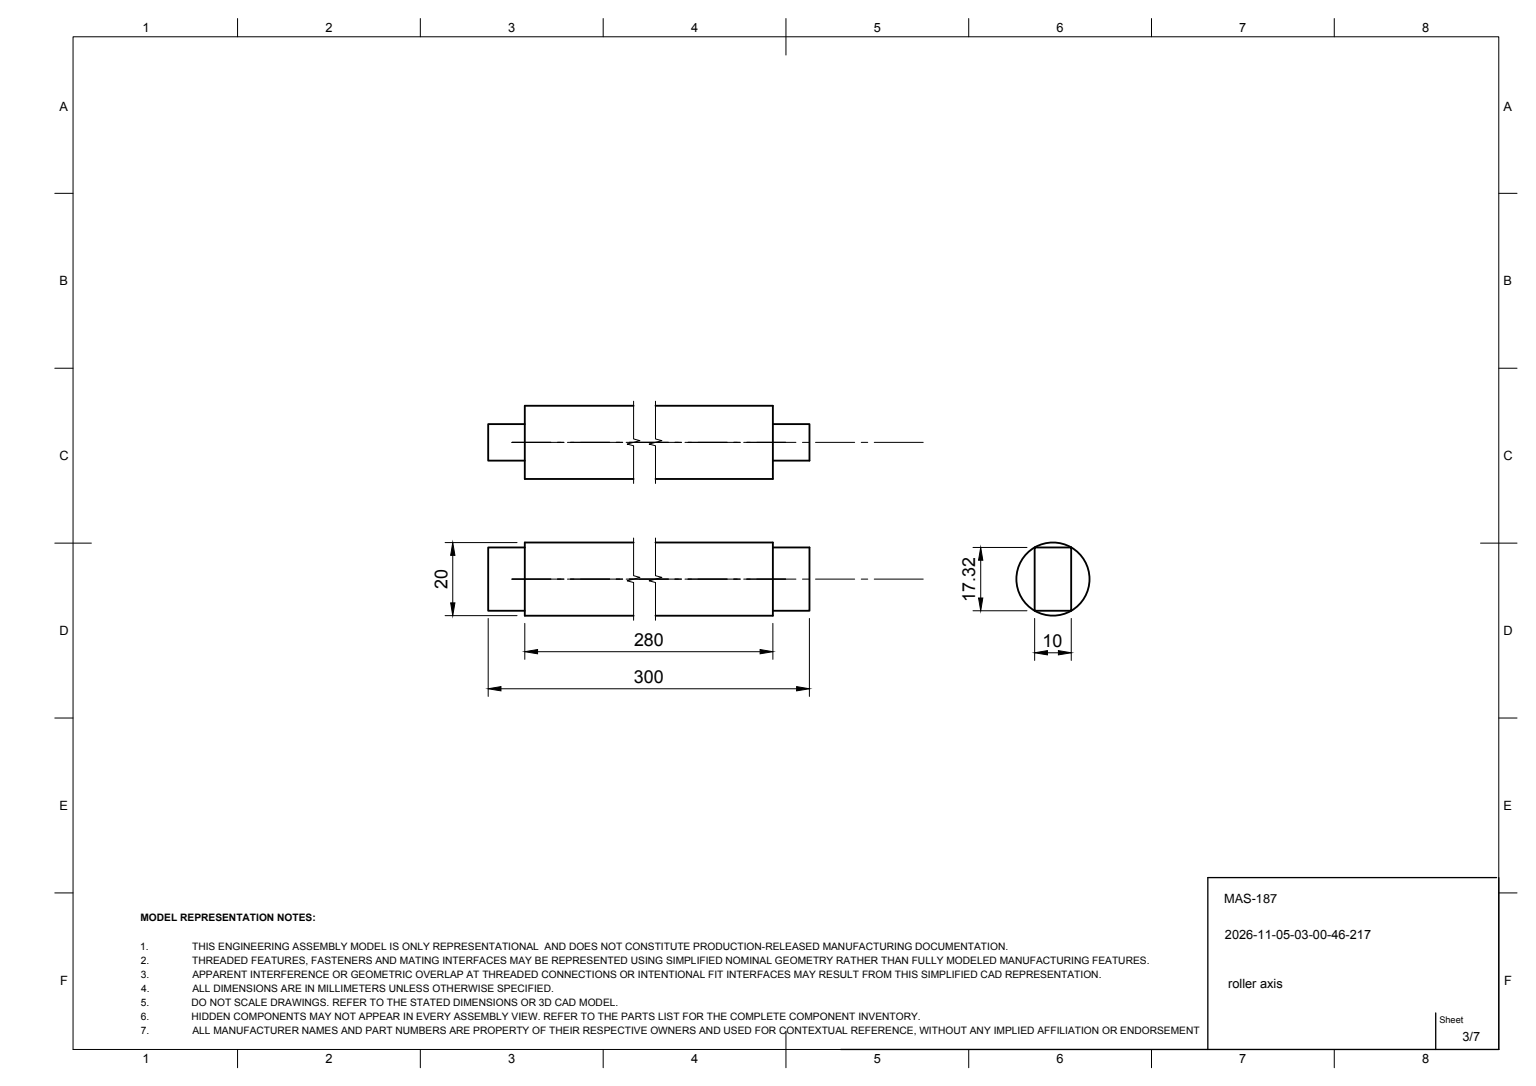
ISO-10303-21;
HEADER;
/* Generated by software containing ST-Developer
 * from STEP Tools, Inc. (www.steptools.com) 
 */

FILE_DESCRIPTION(
/* description */ ('STEP AP214'),
/* implementation_level */ '2;1');

FILE_NAME(
/* name */ 'roller axis.step',
/* time_stamp */ '2026-11-04T19:00:26-08:00',
/* author */ (''),
/* organization */ (''),
/* preprocessor_version */ 'ST-DEVELOPER v20.2',
/* originating_system */ 'Autodesk Translation Framework v15.17.0.0',
/* authorisation */ '');

FILE_SCHEMA (('AUTOMOTIVE_DESIGN { 1 0 10303 214 3 1 1 }'));
ENDSEC;

DATA;
#10=MECHANICAL_DESIGN_GEOMETRIC_PRESENTATION_REPRESENTATION('',(#273),#5689);
#259=SHAPE_REPRESENTATION_RELATIONSHIP('SRR','None',#5760,#266);
#266=ADVANCED_BREP_SHAPE_REPRESENTATION('',(#280),#5684);
#273=STYLED_ITEM('',(#5804),#280);
#280=MANIFOLD_SOLID_BREP('Body1',#2963);
#393=PLANE('',#3168);
#394=PLANE('',#3169);
#395=PLANE('',#3170);
#396=PLANE('',#3171);
#397=PLANE('',#3172);
#398=PLANE('',#3173);
#399=PLANE('',#3174);
#400=PLANE('',#3175);
#401=PLANE('',#3176);
#402=PLANE('',#3177);
#403=PLANE('',#3178);
#404=PLANE('',#3179);
#405=PLANE('',#3180);
#406=PLANE('',#3181);
#407=PLANE('',#3182);
#408=PLANE('',#3183);
#409=PLANE('',#3184);
#410=PLANE('',#3185);
#511=FACE_OUTER_BOUND('',#716,.T.);
#512=FACE_OUTER_BOUND('',#717,.T.);
#513=FACE_OUTER_BOUND('',#718,.T.);
#514=FACE_OUTER_BOUND('',#719,.T.);
#515=FACE_OUTER_BOUND('',#720,.T.);
#516=FACE_OUTER_BOUND('',#721,.T.);
#517=FACE_OUTER_BOUND('',#722,.T.);
#518=FACE_OUTER_BOUND('',#723,.T.);
#519=FACE_OUTER_BOUND('',#724,.T.);
#520=FACE_OUTER_BOUND('',#725,.T.);
#521=FACE_OUTER_BOUND('',#726,.T.);
#522=FACE_OUTER_BOUND('',#727,.T.);
#523=FACE_OUTER_BOUND('',#728,.T.);
#524=FACE_OUTER_BOUND('',#729,.T.);
#525=FACE_OUTER_BOUND('',#730,.T.);
#526=FACE_OUTER_BOUND('',#731,.T.);
#527=FACE_OUTER_BOUND('',#732,.T.);
#528=FACE_OUTER_BOUND('',#733,.T.);
#529=FACE_OUTER_BOUND('',#734,.T.);
#716=EDGE_LOOP('',(#2402,#2403,#2404,#2405,#2406,#2407,#2408,#2409,#2410,
#2411,#2412,#2413));
#717=EDGE_LOOP('',(#2414,#2415,#2416));
#718=EDGE_LOOP('',(#2417,#2418));
#719=EDGE_LOOP('',(#2419,#2420));
#720=EDGE_LOOP('',(#2421,#2422));
#721=EDGE_LOOP('',(#2423,#2424,#2425));
#722=EDGE_LOOP('',(#2426,#2427));
#723=EDGE_LOOP('',(#2428,#2429));
#724=EDGE_LOOP('',(#2430,#2431));
#725=EDGE_LOOP('',(#2432,#2433,#2434,#2435));
#726=EDGE_LOOP('',(#2436,#2437,#2438,#2439));
#727=EDGE_LOOP('',(#2440,#2441,#2442,#2443));
#728=EDGE_LOOP('',(#2444,#2445,#2446,#2447));
#729=EDGE_LOOP('',(#2448,#2449,#2450,#2451));
#730=EDGE_LOOP('',(#2452,#2453,#2454,#2455));
#731=EDGE_LOOP('',(#2456,#2457,#2458,#2459));
#732=EDGE_LOOP('',(#2460,#2461,#2462,#2463));
#733=EDGE_LOOP('',(#2464,#2465,#2466,#2467));
#734=EDGE_LOOP('',(#2468,#2469,#2470,#2471));
#975=LINE('',#4653,#1206);
#976=LINE('',#4667,#1207);
#977=LINE('',#4669,#1208);
#978=LINE('',#4671,#1209);
#979=LINE('',#4673,#1210);
#980=LINE('',#4675,#1211);
#981=LINE('',#4677,#1212);
#982=LINE('',#4679,#1213);
#983=LINE('',#4681,#1214);
#984=LINE('',#4685,#1215);
#985=LINE('',#4687,#1216);
#986=LINE('',#4689,#1217);
#987=LINE('',#4690,#1218);
#988=LINE('',#4692,#1219);
#989=LINE('',#4693,#1220);
#990=LINE('',#4695,#1221);
#991=LINE('',#4697,#1222);
#992=LINE('',#4701,#1223);
#993=LINE('',#4703,#1224);
#994=LINE('',#4704,#1225);
#995=LINE('',#4707,#1226);
#996=LINE('',#4708,#1227);
#997=LINE('',#4711,#1228);
#998=LINE('',#4712,#1229);
#999=LINE('',#4714,#1230);
#1206=VECTOR('',#3756,10.);
#1207=VECTOR('',#3773,1000.);
#1208=VECTOR('',#3776,1000.);
#1209=VECTOR('',#3779,1000.);
#1210=VECTOR('',#3782,1000.);
#1211=VECTOR('',#3785,1000.);
#1212=VECTOR('',#3788,1000.);
#1213=VECTOR('',#3791,1000.);
#1214=VECTOR('',#3794,1000.);
#1215=VECTOR('',#3797,1000.);
#1216=VECTOR('',#3798,1000.);
#1217=VECTOR('',#3799,1000.);
#1218=VECTOR('',#3800,1000.);
#1219=VECTOR('',#3803,1000.);
#1220=VECTOR('',#3804,1000.);
#1221=VECTOR('',#3807,1000.);
#1222=VECTOR('',#3810,1000.);
#1223=VECTOR('',#3815,1000.);
#1224=VECTOR('',#3816,1000.);
#1225=VECTOR('',#3817,1000.);
#1226=VECTOR('',#3820,1000.);
#1227=VECTOR('',#3821,1000.);
#1228=VECTOR('',#3824,1000.);
#1229=VECTOR('',#3825,1000.);
#1230=VECTOR('',#3828,1000.);
#1318=CIRCLE('',#3158,10.);
#1319=CIRCLE('',#3159,10.);
#1320=CIRCLE('',#3160,10.);
#1321=CIRCLE('',#3161,10.);
#1322=CIRCLE('',#3162,10.);
#1323=CIRCLE('',#3163,10.);
#1324=CIRCLE('',#3164,10.);
#1325=CIRCLE('',#3165,10.);
#1326=CIRCLE('',#3166,10.);
#1327=CIRCLE('',#3167,10.);
#1525=VERTEX_POINT('',#4645);
#1526=VERTEX_POINT('',#4646);
#1527=VERTEX_POINT('',#4648);
#1528=VERTEX_POINT('',#4650);
#1529=VERTEX_POINT('',#4652);
#1530=VERTEX_POINT('',#4654);
#1531=VERTEX_POINT('',#4656);
#1532=VERTEX_POINT('',#4658);
#1533=VERTEX_POINT('',#4660);
#1534=VERTEX_POINT('',#4663);
#1535=VERTEX_POINT('',#4683);
#1536=VERTEX_POINT('',#4684);
#1537=VERTEX_POINT('',#4686);
#1538=VERTEX_POINT('',#4688);
#1539=VERTEX_POINT('',#4700);
#1540=VERTEX_POINT('',#4702);
#1541=VERTEX_POINT('',#4706);
#1542=VERTEX_POINT('',#4710);
#1829=EDGE_CURVE('',#1525,#1526,#1318,.T.);
#1830=EDGE_CURVE('',#1526,#1527,#1319,.T.);
#1831=EDGE_CURVE('',#1527,#1528,#1320,.T.);
#1832=EDGE_CURVE('',#1528,#1529,#975,.T.);
#1833=EDGE_CURVE('',#1530,#1529,#1321,.T.);
#1834=EDGE_CURVE('',#1531,#1530,#1322,.T.);
#1835=EDGE_CURVE('',#1532,#1531,#1323,.T.);
#1836=EDGE_CURVE('',#1533,#1532,#1324,.T.);
#1837=EDGE_CURVE('',#1529,#1533,#1325,.T.);
#1838=EDGE_CURVE('',#1528,#1534,#1326,.T.);
#1839=EDGE_CURVE('',#1534,#1525,#1327,.T.);
#1840=EDGE_CURVE('',#1533,#1530,#976,.T.);
#1841=EDGE_CURVE('',#1532,#1533,#977,.T.);
#1842=EDGE_CURVE('',#1531,#1532,#978,.T.);
#1843=EDGE_CURVE('',#1530,#1531,#979,.T.);
#1844=EDGE_CURVE('',#1534,#1527,#980,.T.);
#1845=EDGE_CURVE('',#1525,#1534,#981,.T.);
#1846=EDGE_CURVE('',#1526,#1525,#982,.T.);
#1847=EDGE_CURVE('',#1527,#1526,#983,.T.);
#1848=EDGE_CURVE('',#1535,#1536,#984,.T.);
#1849=EDGE_CURVE('',#1537,#1535,#985,.T.);
#1850=EDGE_CURVE('',#1538,#1537,#986,.T.);
#1851=EDGE_CURVE('',#1536,#1538,#987,.T.);
#1852=EDGE_CURVE('',#1527,#1535,#988,.T.);
#1853=EDGE_CURVE('',#1526,#1537,#989,.T.);
#1854=EDGE_CURVE('',#1525,#1538,#990,.T.);
#1855=EDGE_CURVE('',#1534,#1536,#991,.T.);
#1856=EDGE_CURVE('',#1539,#1533,#992,.T.);
#1857=EDGE_CURVE('',#1540,#1539,#993,.T.);
#1858=EDGE_CURVE('',#1540,#1530,#994,.T.);
#1859=EDGE_CURVE('',#1541,#1532,#995,.T.);
#1860=EDGE_CURVE('',#1539,#1541,#996,.T.);
#1861=EDGE_CURVE('',#1542,#1531,#997,.T.);
#1862=EDGE_CURVE('',#1541,#1542,#998,.T.);
#1863=EDGE_CURVE('',#1542,#1540,#999,.T.);
#2402=ORIENTED_EDGE('',*,*,#1829,.T.);
#2403=ORIENTED_EDGE('',*,*,#1830,.T.);
#2404=ORIENTED_EDGE('',*,*,#1831,.T.);
#2405=ORIENTED_EDGE('',*,*,#1832,.T.);
#2406=ORIENTED_EDGE('',*,*,#1833,.F.);
#2407=ORIENTED_EDGE('',*,*,#1834,.F.);
#2408=ORIENTED_EDGE('',*,*,#1835,.F.);
#2409=ORIENTED_EDGE('',*,*,#1836,.F.);
#2410=ORIENTED_EDGE('',*,*,#1837,.F.);
#2411=ORIENTED_EDGE('',*,*,#1832,.F.);
#2412=ORIENTED_EDGE('',*,*,#1838,.T.);
#2413=ORIENTED_EDGE('',*,*,#1839,.T.);
#2414=ORIENTED_EDGE('',*,*,#1833,.T.);
#2415=ORIENTED_EDGE('',*,*,#1837,.T.);
#2416=ORIENTED_EDGE('',*,*,#1840,.T.);
#2417=ORIENTED_EDGE('',*,*,#1836,.T.);
#2418=ORIENTED_EDGE('',*,*,#1841,.T.);
#2419=ORIENTED_EDGE('',*,*,#1835,.T.);
#2420=ORIENTED_EDGE('',*,*,#1842,.T.);
#2421=ORIENTED_EDGE('',*,*,#1834,.T.);
#2422=ORIENTED_EDGE('',*,*,#1843,.T.);
#2423=ORIENTED_EDGE('',*,*,#1844,.F.);
#2424=ORIENTED_EDGE('',*,*,#1838,.F.);
#2425=ORIENTED_EDGE('',*,*,#1831,.F.);
#2426=ORIENTED_EDGE('',*,*,#1845,.F.);
#2427=ORIENTED_EDGE('',*,*,#1839,.F.);
#2428=ORIENTED_EDGE('',*,*,#1846,.F.);
#2429=ORIENTED_EDGE('',*,*,#1829,.F.);
#2430=ORIENTED_EDGE('',*,*,#1847,.F.);
#2431=ORIENTED_EDGE('',*,*,#1830,.F.);
#2432=ORIENTED_EDGE('',*,*,#1848,.F.);
#2433=ORIENTED_EDGE('',*,*,#1849,.F.);
#2434=ORIENTED_EDGE('',*,*,#1850,.F.);
#2435=ORIENTED_EDGE('',*,*,#1851,.F.);
#2436=ORIENTED_EDGE('',*,*,#1852,.F.);
#2437=ORIENTED_EDGE('',*,*,#1847,.T.);
#2438=ORIENTED_EDGE('',*,*,#1853,.T.);
#2439=ORIENTED_EDGE('',*,*,#1849,.T.);
#2440=ORIENTED_EDGE('',*,*,#1853,.F.);
#2441=ORIENTED_EDGE('',*,*,#1846,.T.);
#2442=ORIENTED_EDGE('',*,*,#1854,.T.);
#2443=ORIENTED_EDGE('',*,*,#1850,.T.);
#2444=ORIENTED_EDGE('',*,*,#1854,.F.);
#2445=ORIENTED_EDGE('',*,*,#1845,.T.);
#2446=ORIENTED_EDGE('',*,*,#1855,.T.);
#2447=ORIENTED_EDGE('',*,*,#1851,.T.);
#2448=ORIENTED_EDGE('',*,*,#1855,.F.);
#2449=ORIENTED_EDGE('',*,*,#1844,.T.);
#2450=ORIENTED_EDGE('',*,*,#1852,.T.);
#2451=ORIENTED_EDGE('',*,*,#1848,.T.);
#2452=ORIENTED_EDGE('',*,*,#1840,.F.);
#2453=ORIENTED_EDGE('',*,*,#1856,.F.);
#2454=ORIENTED_EDGE('',*,*,#1857,.F.);
#2455=ORIENTED_EDGE('',*,*,#1858,.T.);
#2456=ORIENTED_EDGE('',*,*,#1841,.F.);
#2457=ORIENTED_EDGE('',*,*,#1859,.F.);
#2458=ORIENTED_EDGE('',*,*,#1860,.F.);
#2459=ORIENTED_EDGE('',*,*,#1856,.T.);
#2460=ORIENTED_EDGE('',*,*,#1842,.F.);
#2461=ORIENTED_EDGE('',*,*,#1861,.F.);
#2462=ORIENTED_EDGE('',*,*,#1862,.F.);
#2463=ORIENTED_EDGE('',*,*,#1859,.T.);
#2464=ORIENTED_EDGE('',*,*,#1843,.F.);
#2465=ORIENTED_EDGE('',*,*,#1858,.F.);
#2466=ORIENTED_EDGE('',*,*,#1863,.F.);
#2467=ORIENTED_EDGE('',*,*,#1861,.T.);
#2468=ORIENTED_EDGE('',*,*,#1857,.T.);
#2469=ORIENTED_EDGE('',*,*,#1860,.T.);
#2470=ORIENTED_EDGE('',*,*,#1862,.T.);
#2471=ORIENTED_EDGE('',*,*,#1863,.T.);
#2787=CYLINDRICAL_SURFACE('',#3157,10.);
#2871=ADVANCED_FACE('',(#511),#2787,.T.);
#2872=ADVANCED_FACE('',(#512),#393,.T.);
#2873=ADVANCED_FACE('',(#513),#394,.T.);
#2874=ADVANCED_FACE('',(#514),#395,.T.);
#2875=ADVANCED_FACE('',(#515),#396,.T.);
#2876=ADVANCED_FACE('',(#516),#397,.F.);
#2877=ADVANCED_FACE('',(#517),#398,.F.);
#2878=ADVANCED_FACE('',(#518),#399,.F.);
#2879=ADVANCED_FACE('',(#519),#400,.F.);
#2880=ADVANCED_FACE('',(#520),#401,.F.);
#2881=ADVANCED_FACE('',(#521),#402,.F.);
#2882=ADVANCED_FACE('',(#522),#403,.F.);
#2883=ADVANCED_FACE('',(#523),#404,.F.);
#2884=ADVANCED_FACE('',(#524),#405,.F.);
#2885=ADVANCED_FACE('',(#525),#406,.F.);
#2886=ADVANCED_FACE('',(#526),#407,.F.);
#2887=ADVANCED_FACE('',(#527),#408,.F.);
#2888=ADVANCED_FACE('',(#528),#409,.F.);
#2889=ADVANCED_FACE('',(#529),#410,.T.);
#2963=CLOSED_SHELL('',(#2871,#2872,#2873,#2874,#2875,#2876,#2877,#2878,
#2879,#2880,#2881,#2882,#2883,#2884,#2885,#2886,#2887,#2888,#2889));
#3156=AXIS2_PLACEMENT_3D('',#4643,#3746,#3747);
#3157=AXIS2_PLACEMENT_3D('',#4644,#3748,#3749);
#3158=AXIS2_PLACEMENT_3D('',#4647,#3750,#3751);
#3159=AXIS2_PLACEMENT_3D('',#4649,#3752,#3753);
#3160=AXIS2_PLACEMENT_3D('',#4651,#3754,#3755);
#3161=AXIS2_PLACEMENT_3D('',#4655,#3757,#3758);
#3162=AXIS2_PLACEMENT_3D('',#4657,#3759,#3760);
#3163=AXIS2_PLACEMENT_3D('',#4659,#3761,#3762);
#3164=AXIS2_PLACEMENT_3D('',#4661,#3763,#3764);
#3165=AXIS2_PLACEMENT_3D('',#4662,#3765,#3766);
#3166=AXIS2_PLACEMENT_3D('',#4664,#3767,#3768);
#3167=AXIS2_PLACEMENT_3D('',#4665,#3769,#3770);
#3168=AXIS2_PLACEMENT_3D('',#4666,#3771,#3772);
#3169=AXIS2_PLACEMENT_3D('',#4668,#3774,#3775);
#3170=AXIS2_PLACEMENT_3D('',#4670,#3777,#3778);
#3171=AXIS2_PLACEMENT_3D('',#4672,#3780,#3781);
#3172=AXIS2_PLACEMENT_3D('',#4674,#3783,#3784);
#3173=AXIS2_PLACEMENT_3D('',#4676,#3786,#3787);
#3174=AXIS2_PLACEMENT_3D('',#4678,#3789,#3790);
#3175=AXIS2_PLACEMENT_3D('',#4680,#3792,#3793);
#3176=AXIS2_PLACEMENT_3D('',#4682,#3795,#3796);
#3177=AXIS2_PLACEMENT_3D('',#4691,#3801,#3802);
#3178=AXIS2_PLACEMENT_3D('',#4694,#3805,#3806);
#3179=AXIS2_PLACEMENT_3D('',#4696,#3808,#3809);
#3180=AXIS2_PLACEMENT_3D('',#4698,#3811,#3812);
#3181=AXIS2_PLACEMENT_3D('',#4699,#3813,#3814);
#3182=AXIS2_PLACEMENT_3D('',#4705,#3818,#3819);
#3183=AXIS2_PLACEMENT_3D('',#4709,#3822,#3823);
#3184=AXIS2_PLACEMENT_3D('',#4713,#3826,#3827);
#3185=AXIS2_PLACEMENT_3D('',#4715,#3829,#3830);
#3746=DIRECTION('axis',(0.,0.,1.));
#3747=DIRECTION('refdir',(1.,0.,0.));
#3748=DIRECTION('center_axis',(0.,0.,-1.));
#3749=DIRECTION('ref_axis',(-1.,0.,0.));
#3750=DIRECTION('center_axis',(0.,0.,1.));
#3751=DIRECTION('ref_axis',(1.,0.,0.));
#3752=DIRECTION('center_axis',(0.,0.,1.));
#3753=DIRECTION('ref_axis',(1.,0.,0.));
#3754=DIRECTION('center_axis',(0.,0.,1.));
#3755=DIRECTION('ref_axis',(1.,0.,0.));
#3756=DIRECTION('',(0.,0.,1.));
#3757=DIRECTION('center_axis',(0.,0.,1.));
#3758=DIRECTION('ref_axis',(1.,0.,0.));
#3759=DIRECTION('center_axis',(0.,0.,1.));
#3760=DIRECTION('ref_axis',(1.,0.,0.));
#3761=DIRECTION('center_axis',(0.,0.,1.));
#3762=DIRECTION('ref_axis',(1.,0.,0.));
#3763=DIRECTION('center_axis',(0.,0.,1.));
#3764=DIRECTION('ref_axis',(1.,0.,0.));
#3765=DIRECTION('center_axis',(0.,0.,1.));
#3766=DIRECTION('ref_axis',(1.,0.,0.));
#3767=DIRECTION('center_axis',(0.,0.,1.));
#3768=DIRECTION('ref_axis',(1.,0.,0.));
#3769=DIRECTION('center_axis',(0.,0.,1.));
#3770=DIRECTION('ref_axis',(1.,0.,0.));
#3771=DIRECTION('center_axis',(0.,0.,1.));
#3772=DIRECTION('ref_axis',(1.,0.,0.));
#3773=DIRECTION('',(0.,-1.,0.));
#3774=DIRECTION('center_axis',(0.,0.,1.));
#3775=DIRECTION('ref_axis',(1.,0.,0.));
#3776=DIRECTION('',(1.,0.,0.));
#3777=DIRECTION('center_axis',(0.,0.,1.));
#3778=DIRECTION('ref_axis',(1.,0.,0.));
#3779=DIRECTION('',(0.,1.,0.));
#3780=DIRECTION('center_axis',(0.,0.,1.));
#3781=DIRECTION('ref_axis',(1.,0.,0.));
#3782=DIRECTION('',(-1.,0.,0.));
#3783=DIRECTION('center_axis',(0.,0.,1.));
#3784=DIRECTION('ref_axis',(1.,0.,0.));
#3785=DIRECTION('',(0.,-1.,0.));
#3786=DIRECTION('center_axis',(0.,0.,1.));
#3787=DIRECTION('ref_axis',(1.,0.,0.));
#3788=DIRECTION('',(1.,0.,0.));
#3789=DIRECTION('center_axis',(0.,0.,1.));
#3790=DIRECTION('ref_axis',(1.,0.,0.));
#3791=DIRECTION('',(0.,1.,0.));
#3792=DIRECTION('center_axis',(0.,0.,1.));
#3793=DIRECTION('ref_axis',(1.,0.,0.));
#3794=DIRECTION('',(-1.,0.,0.));
#3795=DIRECTION('center_axis',(0.,0.,1.));
#3796=DIRECTION('ref_axis',(1.,0.,0.));
#3797=DIRECTION('',(0.,1.,0.));
#3798=DIRECTION('',(1.,0.,0.));
#3799=DIRECTION('',(0.,-1.,0.));
#3800=DIRECTION('',(-1.,0.,0.));
#3801=DIRECTION('center_axis',(0.,1.,0.));
#3802=DIRECTION('ref_axis',(0.,0.,1.));
#3803=DIRECTION('',(0.,0.,-1.));
#3804=DIRECTION('',(0.,0.,-1.));
#3805=DIRECTION('center_axis',(1.,0.,0.));
#3806=DIRECTION('ref_axis',(0.,0.,-1.));
#3807=DIRECTION('',(0.,0.,-1.));
#3808=DIRECTION('center_axis',(0.,-1.,0.));
#3809=DIRECTION('ref_axis',(0.,0.,-1.));
#3810=DIRECTION('',(0.,0.,-1.));
#3811=DIRECTION('center_axis',(-1.,0.,0.));
#3812=DIRECTION('ref_axis',(0.,0.,1.));
#3813=DIRECTION('center_axis',(-1.,0.,0.));
#3814=DIRECTION('ref_axis',(0.,0.,1.));
#3815=DIRECTION('',(0.,0.,-1.));
#3816=DIRECTION('',(0.,1.,0.));
#3817=DIRECTION('',(0.,0.,-1.));
#3818=DIRECTION('center_axis',(0.,-1.,0.));
#3819=DIRECTION('ref_axis',(0.,0.,-1.));
#3820=DIRECTION('',(0.,0.,-1.));
#3821=DIRECTION('',(-1.,0.,0.));
#3822=DIRECTION('center_axis',(1.,0.,0.));
#3823=DIRECTION('ref_axis',(0.,0.,-1.));
#3824=DIRECTION('',(0.,0.,-1.));
#3825=DIRECTION('',(0.,-1.,0.));
#3826=DIRECTION('center_axis',(0.,1.,0.));
#3827=DIRECTION('ref_axis',(0.,0.,1.));
#3828=DIRECTION('',(1.,0.,0.));
#3829=DIRECTION('center_axis',(0.,0.,1.));
#3830=DIRECTION('ref_axis',(1.,0.,0.));
#4643=CARTESIAN_POINT('',(0.,0.,0.));
#4644=CARTESIAN_POINT('Origin',(0.,0.,140.));
#4645=CARTESIAN_POINT('',(-5.,8.66025403784439,-140.));
#4646=CARTESIAN_POINT('',(-5.,-8.66025403784439,-140.));
#4647=CARTESIAN_POINT('Origin',(0.,0.,-140.));
#4648=CARTESIAN_POINT('',(5.,-8.66025403784439,-140.));
#4649=CARTESIAN_POINT('Origin',(0.,0.,-140.));
#4650=CARTESIAN_POINT('',(10.,-1.22464679914735E-15,-140.));
#4651=CARTESIAN_POINT('Origin',(0.,0.,-140.));
#4652=CARTESIAN_POINT('',(10.,-1.22464679914735E-15,140.));
#4653=CARTESIAN_POINT('',(10.,-1.22464679914735E-15,140.));
#4654=CARTESIAN_POINT('',(5.,-8.66025403784439,140.));
#4655=CARTESIAN_POINT('Origin',(0.,0.,140.));
#4656=CARTESIAN_POINT('',(-5.,-8.66025403784439,140.));
#4657=CARTESIAN_POINT('Origin',(0.,0.,140.));
#4658=CARTESIAN_POINT('',(-5.,8.66025403784439,140.));
#4659=CARTESIAN_POINT('Origin',(0.,0.,140.));
#4660=CARTESIAN_POINT('',(5.,8.66025403784439,140.));
#4661=CARTESIAN_POINT('Origin',(0.,0.,140.));
#4662=CARTESIAN_POINT('Origin',(0.,0.,140.));
#4663=CARTESIAN_POINT('',(4.99999999999999,8.66025403784439,-140.));
#4664=CARTESIAN_POINT('Origin',(0.,0.,-140.));
#4665=CARTESIAN_POINT('Origin',(0.,0.,-140.));
#4666=CARTESIAN_POINT('Origin',(0.,0.,140.));
#4667=CARTESIAN_POINT('',(5.,0.,140.));
#4668=CARTESIAN_POINT('Origin',(0.,0.,140.));
#4669=CARTESIAN_POINT('',(0.,8.66025403784439,140.));
#4670=CARTESIAN_POINT('Origin',(0.,0.,140.));
#4671=CARTESIAN_POINT('',(-5.,0.,140.));
#4672=CARTESIAN_POINT('Origin',(0.,0.,140.));
#4673=CARTESIAN_POINT('',(0.,-8.66025403784439,140.));
#4674=CARTESIAN_POINT('Origin',(0.,0.,-140.));
#4675=CARTESIAN_POINT('',(5.,0.,-140.));
#4676=CARTESIAN_POINT('Origin',(0.,0.,-140.));
#4677=CARTESIAN_POINT('',(0.,8.66025403784439,-140.));
#4678=CARTESIAN_POINT('Origin',(0.,0.,-140.));
#4679=CARTESIAN_POINT('',(-5.,0.,-140.));
#4680=CARTESIAN_POINT('Origin',(0.,0.,-140.));
#4681=CARTESIAN_POINT('',(0.,-8.66025403784439,-140.));
#4682=CARTESIAN_POINT('Origin',(0.,0.,-150.));
#4683=CARTESIAN_POINT('',(5.,-8.66025403784439,-150.));
#4684=CARTESIAN_POINT('',(5.,8.66025403784439,-150.));
#4685=CARTESIAN_POINT('',(5.,8.66025403784439,-150.));
#4686=CARTESIAN_POINT('',(-5.,-8.66025403784439,-150.));
#4687=CARTESIAN_POINT('',(-5.,-8.66025403784439,-150.));
#4688=CARTESIAN_POINT('',(-5.,8.66025403784439,-150.));
#4689=CARTESIAN_POINT('',(-5.,8.66025403784439,-150.));
#4690=CARTESIAN_POINT('',(-5.,8.66025403784439,-150.));
#4691=CARTESIAN_POINT('Origin',(-5.,-8.66025403784439,150.));
#4692=CARTESIAN_POINT('',(5.,-8.66025403784439,150.));
#4693=CARTESIAN_POINT('',(-5.,-8.66025403784439,150.));
#4694=CARTESIAN_POINT('Origin',(-5.,8.66025403784439,150.));
#4695=CARTESIAN_POINT('',(-5.,8.66025403784439,150.));
#4696=CARTESIAN_POINT('Origin',(-5.,8.66025403784439,150.));
#4697=CARTESIAN_POINT('',(5.,8.66025403784439,150.));
#4698=CARTESIAN_POINT('Origin',(5.,8.66025403784439,150.));
#4699=CARTESIAN_POINT('Origin',(5.,8.66025403784439,150.));
#4700=CARTESIAN_POINT('',(5.,8.66025403784439,150.));
#4701=CARTESIAN_POINT('',(5.,8.66025403784439,150.));
#4702=CARTESIAN_POINT('',(5.,-8.66025403784439,150.));
#4703=CARTESIAN_POINT('',(5.,8.66025403784439,150.));
#4704=CARTESIAN_POINT('',(5.,-8.66025403784439,150.));
#4705=CARTESIAN_POINT('Origin',(-5.,8.66025403784439,150.));
#4706=CARTESIAN_POINT('',(-5.,8.66025403784439,150.));
#4707=CARTESIAN_POINT('',(-5.,8.66025403784439,150.));
#4708=CARTESIAN_POINT('',(-5.,8.66025403784439,150.));
#4709=CARTESIAN_POINT('Origin',(-5.,8.66025403784439,150.));
#4710=CARTESIAN_POINT('',(-5.,-8.66025403784439,150.));
#4711=CARTESIAN_POINT('',(-5.,-8.66025403784439,150.));
#4712=CARTESIAN_POINT('',(-5.,8.66025403784439,150.));
#4713=CARTESIAN_POINT('Origin',(-5.,-8.66025403784439,150.));
#4714=CARTESIAN_POINT('',(-5.,-8.66025403784439,150.));
#4715=CARTESIAN_POINT('Origin',(0.,0.,150.));
#5675=UNCERTAINTY_MEASURE_WITH_UNIT(LENGTH_MEASURE(0.01),#5690,
'DISTANCE_ACCURACY_VALUE',
'Maximum model space distance between geometric entities at asserted c
onnectivities');
#5680=UNCERTAINTY_MEASURE_WITH_UNIT(LENGTH_MEASURE(0.01),#5690,
'DISTANCE_ACCURACY_VALUE',
'Maximum model space distance between geometric entities at asserted c
onnectivities');
#5684=(
GEOMETRIC_REPRESENTATION_CONTEXT(3)
GLOBAL_UNCERTAINTY_ASSIGNED_CONTEXT((#5675))
GLOBAL_UNIT_ASSIGNED_CONTEXT((#5690,#5692,#5693))
REPRESENTATION_CONTEXT('','3D')
);
#5689=(
GEOMETRIC_REPRESENTATION_CONTEXT(3)
GLOBAL_UNCERTAINTY_ASSIGNED_CONTEXT((#5680))
GLOBAL_UNIT_ASSIGNED_CONTEXT((#5690,#5692,#5693))
REPRESENTATION_CONTEXT('','3D')
);
#5690=(
LENGTH_UNIT()
NAMED_UNIT(*)
SI_UNIT(.MILLI.,.METRE.)
);
#5692=(
NAMED_UNIT(*)
PLANE_ANGLE_UNIT()
SI_UNIT($,.RADIAN.)
);
#5693=(
NAMED_UNIT(*)
SI_UNIT($,.STERADIAN.)
SOLID_ANGLE_UNIT()
);
#5697=SHAPE_DEFINITION_REPRESENTATION(#5705,#5760);
#5705=PRODUCT_DEFINITION_SHAPE('',$,#5769);
#5760=SHAPE_REPRESENTATION('',(#3156),#5684);
#5765=PRODUCT_DEFINITION_CONTEXT('part definition',#5791,'design');
#5769=PRODUCT_DEFINITION('roller axis','roller axis',#5777,#5765);
#5777=PRODUCT_DEFINITION_FORMATION('',$,#5796);
#5791=APPLICATION_CONTEXT(
'Core Data for Automotive Mechanical Design Process');
#5792=PRODUCT_CONTEXT('part definition',#5791,'mechanical');
#5796=PRODUCT('roller axis','roller axis',$,(#5792));
#5804=PRESENTATION_STYLE_ASSIGNMENT((#5810));
#5810=SURFACE_STYLE_USAGE(.BOTH.,#5816);
#5816=SURFACE_SIDE_STYLE('',(#5822));
#5822=SURFACE_STYLE_FILL_AREA(#5828);
#5828=FILL_AREA_STYLE('Opaque(61,176,222)',(#5834));
#5834=FILL_AREA_STYLE_COLOUR('Opaque(61,176,222)',#5840);
#5840=COLOUR_RGB('Opaque(61,176,222)',0.23921568627451,0.690196078431373,
0.870588235294118);
ENDSEC;
END-ISO-10303-21;
